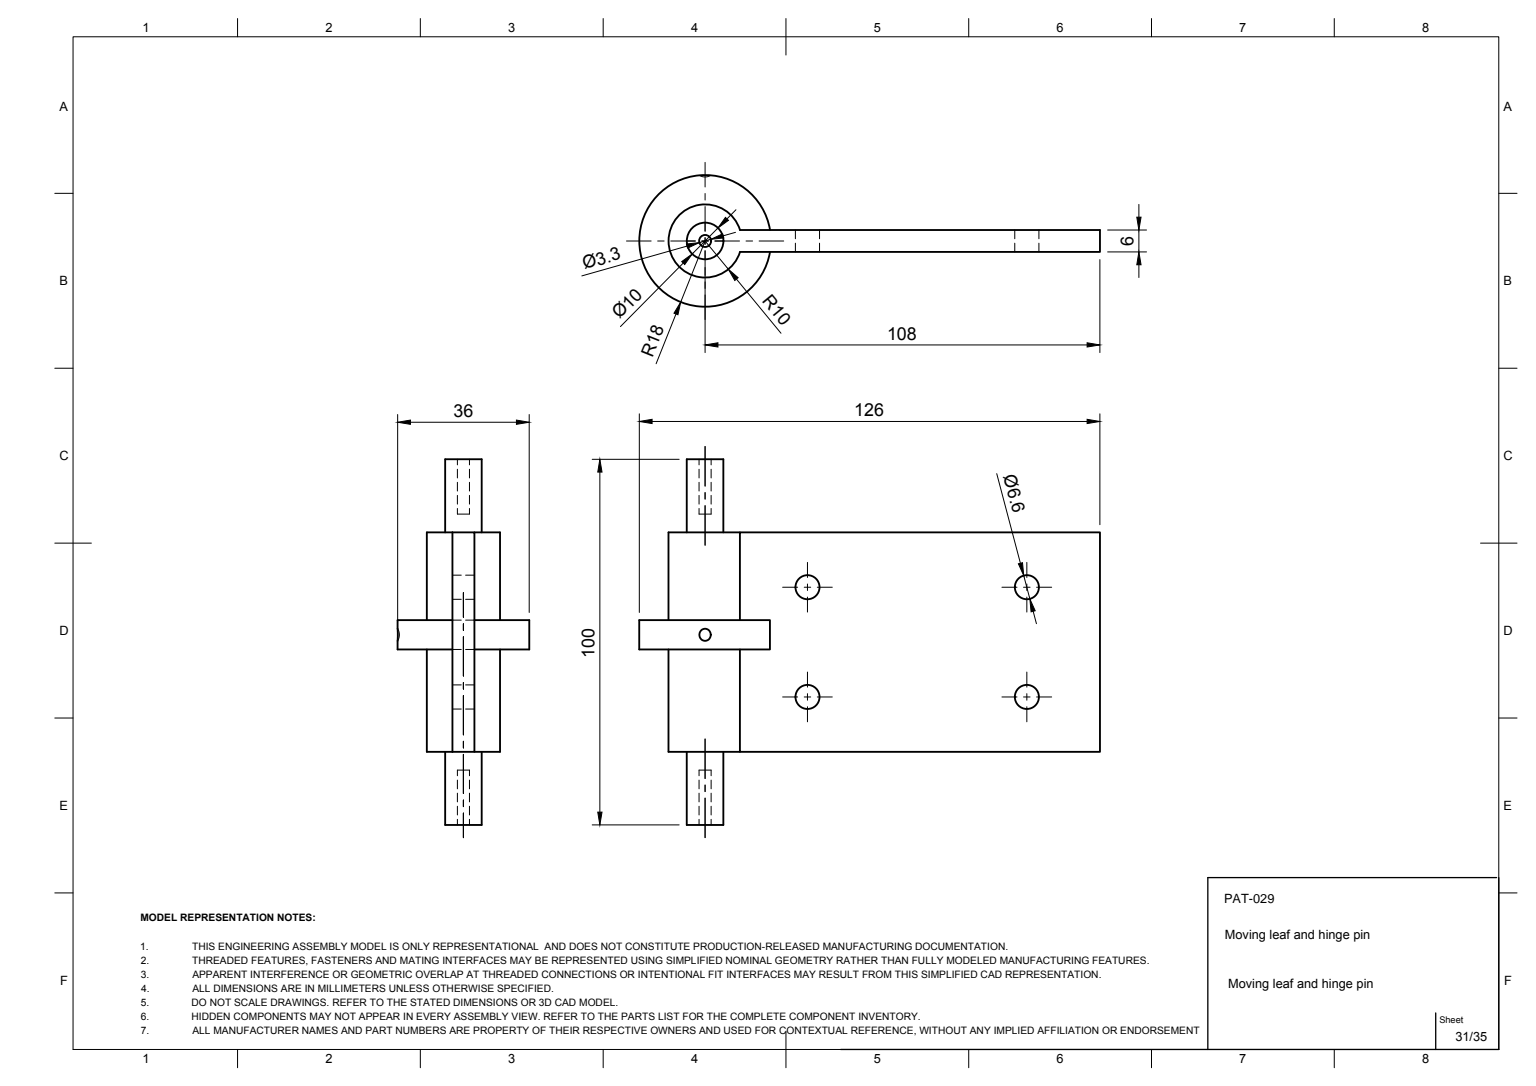
ISO-10303-21;
HEADER;
/* Generated by software containing ST-Developer
 * from STEP Tools, Inc. (www.steptools.com) 
 */

FILE_DESCRIPTION(
/* description */ ('Door-style hinge test fixture with detent'),
/* implementation_level */ '2;1');

FILE_NAME(
/* name */ 'Moving leaf and hinge pin.step',
/* time_stamp */ '2026-10-28T03:24:57-07:00',
/* author */ (''),
/* organization */ (''),
/* preprocessor_version */ 'ST-DEVELOPER v20.2',
/* originating_system */ 'Autodesk Translation Framework v15.17.0.0',
/* authorisation */ '');

FILE_SCHEMA (('AUTOMOTIVE_DESIGN { 1 0 10303 214 3 1 1 }'));
ENDSEC;

DATA;
#10=MECHANICAL_DESIGN_GEOMETRIC_PRESENTATION_REPRESENTATION('',(#356),#9813);
#240=B_SPLINE_CURVE_WITH_KNOTS('',3,(#9473,#9474,#9475,#9476,#9477,#9478,
#9479,#9480,#9481,#9482,#9483,#9484,#9485,#9486,#9487,#9488,#9489,#9490,
#9491,#9492,#9493,#9494,#9495,#9496,#9497,#9498,#9499,#9500,#9501,#9502,
#9503,#9504,#9505,#9506,#9507,#9508,#9509,#9510,#9511,#9512,#9513,#9514),
 .UNSPECIFIED.,.T.,.F.,(4,2,2,2,2,2,2,2,2,2,2,2,2,2,2,2,2,2,2,2,4),(0.,
0.0839475318916269,0.12592129783744,0.167895063783254,0.205982250035365,
0.244069436287477,0.282156622539588,0.320243808791699,0.362217574737513,
0.404191340683327,0.488138872574954,0.572086404466582,0.614060170412395,
0.656033936358209,0.694121122610321,0.732208308862432,0.770295495114543,
0.808382681366655,0.850356447312468,0.892330213258282,0.976277745149909),
 .UNSPECIFIED.);
#259=SPHERICAL_SURFACE('',#5643,0.3);
#285=SHAPE_REPRESENTATION_RELATIONSHIP('SRR','None',#9964,#316);
#316=ADVANCED_BREP_SHAPE_REPRESENTATION('',(#394),#9807);
#356=STYLED_ITEM('',(#10183),#394);
#394=MANIFOLD_SOLID_BREP('Body1',#4789);
#478=FACE_BOUND('',#1263,.T.);
#479=FACE_BOUND('',#1266,.T.);
#480=FACE_BOUND('',#1267,.T.);
#481=FACE_BOUND('',#1268,.T.);
#482=FACE_BOUND('',#1269,.T.);
#483=FACE_BOUND('',#1276,.T.);
#484=FACE_BOUND('',#1277,.T.);
#485=FACE_BOUND('',#1278,.T.);
#486=FACE_BOUND('',#1279,.T.);
#487=FACE_BOUND('',#1283,.T.);
#488=FACE_BOUND('',#1285,.T.);
#489=FACE_BOUND('',#1289,.T.);
#490=FACE_BOUND('',#1291,.T.);
#633=PLANE('',#5638);
#634=PLANE('',#5642);
#635=PLANE('',#5644);
#636=PLANE('',#5649);
#637=PLANE('',#5651);
#638=PLANE('',#5666);
#639=PLANE('',#5667);
#640=PLANE('',#5670);
#641=PLANE('',#5672);
#642=PLANE('',#5678);
#643=PLANE('',#5679);
#892=FACE_OUTER_BOUND('',#1256,.T.);
#893=FACE_OUTER_BOUND('',#1257,.T.);
#894=FACE_OUTER_BOUND('',#1258,.T.);
#895=FACE_OUTER_BOUND('',#1259,.T.);
#896=FACE_OUTER_BOUND('',#1260,.T.);
#897=FACE_OUTER_BOUND('',#1261,.T.);
#898=FACE_OUTER_BOUND('',#1262,.T.);
#899=FACE_OUTER_BOUND('',#1264,.T.);
#900=FACE_OUTER_BOUND('',#1265,.T.);
#901=FACE_OUTER_BOUND('',#1270,.T.);
#902=FACE_OUTER_BOUND('',#1271,.T.);
#903=FACE_OUTER_BOUND('',#1272,.T.);
#904=FACE_OUTER_BOUND('',#1273,.T.);
#905=FACE_OUTER_BOUND('',#1274,.T.);
#906=FACE_OUTER_BOUND('',#1275,.T.);
#907=FACE_OUTER_BOUND('',#1280,.T.);
#908=FACE_OUTER_BOUND('',#1281,.T.);
#909=FACE_OUTER_BOUND('',#1282,.T.);
#910=FACE_OUTER_BOUND('',#1284,.T.);
#911=FACE_OUTER_BOUND('',#1286,.T.);
#912=FACE_OUTER_BOUND('',#1287,.T.);
#913=FACE_OUTER_BOUND('',#1288,.T.);
#914=FACE_OUTER_BOUND('',#1290,.T.);
#1256=EDGE_LOOP('',(#4171,#4172,#4173,#4174));
#1257=EDGE_LOOP('',(#4175));
#1258=EDGE_LOOP('',(#4176,#4177,#4178,#4179));
#1259=EDGE_LOOP('',(#4180));
#1260=EDGE_LOOP('',(#4181));
#1261=EDGE_LOOP('',(#4182,#4183,#4184,#4185));
#1262=EDGE_LOOP('',(#4186,#4187,#4188,#4189));
#1263=EDGE_LOOP('',(#4190));
#1264=EDGE_LOOP('',(#4191,#4192,#4193,#4194));
#1265=EDGE_LOOP('',(#4195,#4196,#4197,#4198,#4199,#4200,#4201,#4202));
#1266=EDGE_LOOP('',(#4203));
#1267=EDGE_LOOP('',(#4204));
#1268=EDGE_LOOP('',(#4205));
#1269=EDGE_LOOP('',(#4206));
#1270=EDGE_LOOP('',(#4207,#4208,#4209,#4210));
#1271=EDGE_LOOP('',(#4211,#4212,#4213,#4214));
#1272=EDGE_LOOP('',(#4215,#4216,#4217,#4218));
#1273=EDGE_LOOP('',(#4219,#4220,#4221,#4222));
#1274=EDGE_LOOP('',(#4223,#4224,#4225,#4226));
#1275=EDGE_LOOP('',(#4227,#4228,#4229,#4230,#4231,#4232,#4233,#4234));
#1276=EDGE_LOOP('',(#4235));
#1277=EDGE_LOOP('',(#4236));
#1278=EDGE_LOOP('',(#4237));
#1279=EDGE_LOOP('',(#4238));
#1280=EDGE_LOOP('',(#4239,#4240,#4241,#4242));
#1281=EDGE_LOOP('',(#4243,#4244,#4245,#4246));
#1282=EDGE_LOOP('',(#4247,#4248,#4249,#4250));
#1283=EDGE_LOOP('',(#4251));
#1284=EDGE_LOOP('',(#4252,#4253,#4254,#4255));
#1285=EDGE_LOOP('',(#4256));
#1286=EDGE_LOOP('',(#4257,#4258,#4259,#4260));
#1287=EDGE_LOOP('',(#4261,#4262,#4263,#4264));
#1288=EDGE_LOOP('',(#4265));
#1289=EDGE_LOOP('',(#4266));
#1290=EDGE_LOOP('',(#4267));
#1291=EDGE_LOOP('',(#4268));
#1596=LINE('',#9461,#1916);
#1597=LINE('',#9468,#1917);
#1598=LINE('',#9518,#1918);
#1599=LINE('',#9522,#1919);
#1600=LINE('',#9526,#1920);
#1601=LINE('',#9528,#1921);
#1602=LINE('',#9532,#1922);
#1603=LINE('',#9534,#1923);
#1604=LINE('',#9538,#1924);
#1605=LINE('',#9540,#1925);
#1606=LINE('',#9542,#1926);
#1607=LINE('',#9544,#1927);
#1608=LINE('',#9545,#1928);
#1609=LINE('',#9556,#1929);
#1610=LINE('',#9560,#1930);
#1611=LINE('',#9564,#1931);
#1612=LINE('',#9568,#1932);
#1613=LINE('',#9572,#1933);
#1614=LINE('',#9576,#1934);
#1615=LINE('',#9578,#1935);
#1616=LINE('',#9580,#1936);
#1617=LINE('',#9581,#1937);
#1618=LINE('',#9583,#1938);
#1619=LINE('',#9584,#1939);
#1620=LINE('',#9595,#1940);
#1621=LINE('',#9600,#1941);
#1916=VECTOR('',#7011,0.165);
#1917=VECTOR('',#7020,0.165);
#1918=VECTOR('',#7029,1.);
#1919=VECTOR('',#7032,1.);
#1920=VECTOR('',#7037,1.);
#1921=VECTOR('',#7038,1.);
#1922=VECTOR('',#7043,1.);
#1923=VECTOR('',#7044,1.);
#1924=VECTOR('',#7049,1.);
#1925=VECTOR('',#7050,1.);
#1926=VECTOR('',#7051,1.);
#1927=VECTOR('',#7052,1.);
#1928=VECTOR('',#7053,1.);
#1929=VECTOR('',#7064,1.);
#1930=VECTOR('',#7069,0.33);
#1931=VECTOR('',#7074,0.33);
#1932=VECTOR('',#7079,0.33);
#1933=VECTOR('',#7084,0.33);
#1934=VECTOR('',#7089,1.);
#1935=VECTOR('',#7090,1.);
#1936=VECTOR('',#7091,1.);
#1937=VECTOR('',#7092,1.);
#1938=VECTOR('',#7095,1.);
#1939=VECTOR('',#7096,1.);
#1940=VECTOR('',#7111,0.5);
#1941=VECTOR('',#7118,0.5);
#2175=CIRCLE('',#5636,0.165);
#2176=CIRCLE('',#5637,0.165);
#2177=CIRCLE('',#5640,0.165);
#2178=CIRCLE('',#5641,0.165);
#2179=CIRCLE('',#5645,1.);
#2180=CIRCLE('',#5646,1.8);
#2181=CIRCLE('',#5648,1.8);
#2182=CIRCLE('',#5650,1.);
#2183=CIRCLE('',#5652,0.33);
#2184=CIRCLE('',#5653,0.33);
#2185=CIRCLE('',#5654,0.33);
#2186=CIRCLE('',#5655,0.33);
#2187=CIRCLE('',#5657,1.);
#2188=CIRCLE('',#5659,0.33);
#2189=CIRCLE('',#5661,0.33);
#2190=CIRCLE('',#5663,0.33);
#2191=CIRCLE('',#5665,0.33);
#2192=CIRCLE('',#5669,1.);
#2193=CIRCLE('',#5671,0.5);
#2194=CIRCLE('',#5673,0.5);
#2195=CIRCLE('',#5675,0.5);
#2196=CIRCLE('',#5677,0.5);
#2551=VERTEX_POINT('',#9458);
#2552=VERTEX_POINT('',#9460);
#2553=VERTEX_POINT('',#9465);
#2554=VERTEX_POINT('',#9467);
#2555=VERTEX_POINT('',#9472);
#2556=VERTEX_POINT('',#9516);
#2557=VERTEX_POINT('',#9517);
#2558=VERTEX_POINT('',#9519);
#2559=VERTEX_POINT('',#9521);
#2560=VERTEX_POINT('',#9525);
#2561=VERTEX_POINT('',#9527);
#2562=VERTEX_POINT('',#9531);
#2563=VERTEX_POINT('',#9533);
#2564=VERTEX_POINT('',#9537);
#2565=VERTEX_POINT('',#9539);
#2566=VERTEX_POINT('',#9541);
#2567=VERTEX_POINT('',#9543);
#2568=VERTEX_POINT('',#9546);
#2569=VERTEX_POINT('',#9548);
#2570=VERTEX_POINT('',#9550);
#2571=VERTEX_POINT('',#9552);
#2572=VERTEX_POINT('',#9555);
#2573=VERTEX_POINT('',#9559);
#2574=VERTEX_POINT('',#9563);
#2575=VERTEX_POINT('',#9567);
#2576=VERTEX_POINT('',#9571);
#2577=VERTEX_POINT('',#9575);
#2578=VERTEX_POINT('',#9577);
#2579=VERTEX_POINT('',#9579);
#2580=VERTEX_POINT('',#9588);
#2581=VERTEX_POINT('',#9591);
#2582=VERTEX_POINT('',#9594);
#2583=VERTEX_POINT('',#9598);
#3102=EDGE_CURVE('',#2551,#2551,#2175,.T.);
#3103=EDGE_CURVE('',#2551,#2552,#1596,.T.);
#3104=EDGE_CURVE('',#2552,#2552,#2176,.T.);
#3105=EDGE_CURVE('',#2553,#2553,#2177,.T.);
#3106=EDGE_CURVE('',#2553,#2554,#1597,.T.);
#3107=EDGE_CURVE('',#2554,#2554,#2178,.T.);
#3108=EDGE_CURVE('',#2555,#2555,#240,.T.);
#3109=EDGE_CURVE('',#2556,#2557,#1598,.T.);
#3110=EDGE_CURVE('',#2558,#2556,#2179,.T.);
#3111=EDGE_CURVE('',#2559,#2558,#1599,.T.);
#3112=EDGE_CURVE('',#2559,#2557,#2180,.T.);
#3113=EDGE_CURVE('',#2557,#2560,#1600,.T.);
#3114=EDGE_CURVE('',#2561,#2559,#1601,.T.);
#3115=EDGE_CURVE('',#2561,#2560,#2181,.T.);
#3116=EDGE_CURVE('',#2560,#2562,#1602,.T.);
#3117=EDGE_CURVE('',#2563,#2561,#1603,.T.);
#3118=EDGE_CURVE('',#2562,#2563,#2182,.T.);
#3119=EDGE_CURVE('',#2564,#2562,#1604,.T.);
#3120=EDGE_CURVE('',#2564,#2565,#1605,.T.);
#3121=EDGE_CURVE('',#2565,#2566,#1606,.T.);
#3122=EDGE_CURVE('',#2567,#2566,#1607,.T.);
#3123=EDGE_CURVE('',#2556,#2567,#1608,.T.);
#3124=EDGE_CURVE('',#2568,#2568,#2183,.T.);
#3125=EDGE_CURVE('',#2569,#2569,#2184,.T.);
#3126=EDGE_CURVE('',#2570,#2570,#2185,.T.);
#3127=EDGE_CURVE('',#2571,#2571,#2186,.T.);
#3128=EDGE_CURVE('',#2563,#2572,#1609,.T.);
#3129=EDGE_CURVE('',#2572,#2564,#2187,.T.);
#3130=EDGE_CURVE('',#2571,#2573,#1610,.T.);
#3131=EDGE_CURVE('',#2573,#2573,#2188,.T.);
#3132=EDGE_CURVE('',#2570,#2574,#1611,.T.);
#3133=EDGE_CURVE('',#2574,#2574,#2189,.T.);
#3134=EDGE_CURVE('',#2569,#2575,#1612,.T.);
#3135=EDGE_CURVE('',#2575,#2575,#2190,.T.);
#3136=EDGE_CURVE('',#2568,#2576,#1613,.T.);
#3137=EDGE_CURVE('',#2576,#2576,#2191,.T.);
#3138=EDGE_CURVE('',#2577,#2558,#1614,.T.);
#3139=EDGE_CURVE('',#2578,#2577,#1615,.T.);
#3140=EDGE_CURVE('',#2579,#2578,#1616,.T.);
#3141=EDGE_CURVE('',#2579,#2572,#1617,.T.);
#3142=EDGE_CURVE('',#2565,#2579,#1618,.T.);
#3143=EDGE_CURVE('',#2566,#2578,#1619,.T.);
#3144=EDGE_CURVE('',#2577,#2567,#2192,.T.);
#3145=EDGE_CURVE('',#2580,#2580,#2193,.T.);
#3146=EDGE_CURVE('',#2581,#2581,#2194,.T.);
#3147=EDGE_CURVE('',#2580,#2582,#1620,.T.);
#3148=EDGE_CURVE('',#2582,#2582,#2195,.T.);
#3149=EDGE_CURVE('',#2583,#2583,#2196,.T.);
#3150=EDGE_CURVE('',#2583,#2581,#1621,.T.);
#4171=ORIENTED_EDGE('',*,*,#3102,.F.);
#4172=ORIENTED_EDGE('',*,*,#3103,.T.);
#4173=ORIENTED_EDGE('',*,*,#3104,.F.);
#4174=ORIENTED_EDGE('',*,*,#3103,.F.);
#4175=ORIENTED_EDGE('',*,*,#3102,.T.);
#4176=ORIENTED_EDGE('',*,*,#3105,.F.);
#4177=ORIENTED_EDGE('',*,*,#3106,.T.);
#4178=ORIENTED_EDGE('',*,*,#3107,.T.);
#4179=ORIENTED_EDGE('',*,*,#3106,.F.);
#4180=ORIENTED_EDGE('',*,*,#3107,.F.);
#4181=ORIENTED_EDGE('',*,*,#3108,.F.);
#4182=ORIENTED_EDGE('',*,*,#3109,.F.);
#4183=ORIENTED_EDGE('',*,*,#3110,.F.);
#4184=ORIENTED_EDGE('',*,*,#3111,.F.);
#4185=ORIENTED_EDGE('',*,*,#3112,.T.);
#4186=ORIENTED_EDGE('',*,*,#3113,.F.);
#4187=ORIENTED_EDGE('',*,*,#3112,.F.);
#4188=ORIENTED_EDGE('',*,*,#3114,.F.);
#4189=ORIENTED_EDGE('',*,*,#3115,.T.);
#4190=ORIENTED_EDGE('',*,*,#3108,.T.);
#4191=ORIENTED_EDGE('',*,*,#3116,.F.);
#4192=ORIENTED_EDGE('',*,*,#3115,.F.);
#4193=ORIENTED_EDGE('',*,*,#3117,.F.);
#4194=ORIENTED_EDGE('',*,*,#3118,.F.);
#4195=ORIENTED_EDGE('',*,*,#3109,.T.);
#4196=ORIENTED_EDGE('',*,*,#3113,.T.);
#4197=ORIENTED_EDGE('',*,*,#3116,.T.);
#4198=ORIENTED_EDGE('',*,*,#3119,.F.);
#4199=ORIENTED_EDGE('',*,*,#3120,.T.);
#4200=ORIENTED_EDGE('',*,*,#3121,.T.);
#4201=ORIENTED_EDGE('',*,*,#3122,.F.);
#4202=ORIENTED_EDGE('',*,*,#3123,.F.);
#4203=ORIENTED_EDGE('',*,*,#3124,.T.);
#4204=ORIENTED_EDGE('',*,*,#3125,.T.);
#4205=ORIENTED_EDGE('',*,*,#3126,.T.);
#4206=ORIENTED_EDGE('',*,*,#3127,.T.);
#4207=ORIENTED_EDGE('',*,*,#3118,.T.);
#4208=ORIENTED_EDGE('',*,*,#3128,.T.);
#4209=ORIENTED_EDGE('',*,*,#3129,.T.);
#4210=ORIENTED_EDGE('',*,*,#3119,.T.);
#4211=ORIENTED_EDGE('',*,*,#3127,.F.);
#4212=ORIENTED_EDGE('',*,*,#3130,.T.);
#4213=ORIENTED_EDGE('',*,*,#3131,.F.);
#4214=ORIENTED_EDGE('',*,*,#3130,.F.);
#4215=ORIENTED_EDGE('',*,*,#3126,.F.);
#4216=ORIENTED_EDGE('',*,*,#3132,.T.);
#4217=ORIENTED_EDGE('',*,*,#3133,.F.);
#4218=ORIENTED_EDGE('',*,*,#3132,.F.);
#4219=ORIENTED_EDGE('',*,*,#3125,.F.);
#4220=ORIENTED_EDGE('',*,*,#3134,.T.);
#4221=ORIENTED_EDGE('',*,*,#3135,.F.);
#4222=ORIENTED_EDGE('',*,*,#3134,.F.);
#4223=ORIENTED_EDGE('',*,*,#3124,.F.);
#4224=ORIENTED_EDGE('',*,*,#3136,.T.);
#4225=ORIENTED_EDGE('',*,*,#3137,.F.);
#4226=ORIENTED_EDGE('',*,*,#3136,.F.);
#4227=ORIENTED_EDGE('',*,*,#3111,.T.);
#4228=ORIENTED_EDGE('',*,*,#3138,.F.);
#4229=ORIENTED_EDGE('',*,*,#3139,.F.);
#4230=ORIENTED_EDGE('',*,*,#3140,.F.);
#4231=ORIENTED_EDGE('',*,*,#3141,.T.);
#4232=ORIENTED_EDGE('',*,*,#3128,.F.);
#4233=ORIENTED_EDGE('',*,*,#3117,.T.);
#4234=ORIENTED_EDGE('',*,*,#3114,.T.);
#4235=ORIENTED_EDGE('',*,*,#3131,.T.);
#4236=ORIENTED_EDGE('',*,*,#3133,.T.);
#4237=ORIENTED_EDGE('',*,*,#3135,.T.);
#4238=ORIENTED_EDGE('',*,*,#3137,.T.);
#4239=ORIENTED_EDGE('',*,*,#3142,.T.);
#4240=ORIENTED_EDGE('',*,*,#3140,.T.);
#4241=ORIENTED_EDGE('',*,*,#3143,.F.);
#4242=ORIENTED_EDGE('',*,*,#3121,.F.);
#4243=ORIENTED_EDGE('',*,*,#3110,.T.);
#4244=ORIENTED_EDGE('',*,*,#3123,.T.);
#4245=ORIENTED_EDGE('',*,*,#3144,.F.);
#4246=ORIENTED_EDGE('',*,*,#3138,.T.);
#4247=ORIENTED_EDGE('',*,*,#3129,.F.);
#4248=ORIENTED_EDGE('',*,*,#3141,.F.);
#4249=ORIENTED_EDGE('',*,*,#3142,.F.);
#4250=ORIENTED_EDGE('',*,*,#3120,.F.);
#4251=ORIENTED_EDGE('',*,*,#3145,.F.);
#4252=ORIENTED_EDGE('',*,*,#3144,.T.);
#4253=ORIENTED_EDGE('',*,*,#3122,.T.);
#4254=ORIENTED_EDGE('',*,*,#3143,.T.);
#4255=ORIENTED_EDGE('',*,*,#3139,.T.);
#4256=ORIENTED_EDGE('',*,*,#3146,.F.);
#4257=ORIENTED_EDGE('',*,*,#3145,.T.);
#4258=ORIENTED_EDGE('',*,*,#3147,.T.);
#4259=ORIENTED_EDGE('',*,*,#3148,.T.);
#4260=ORIENTED_EDGE('',*,*,#3147,.F.);
#4261=ORIENTED_EDGE('',*,*,#3149,.F.);
#4262=ORIENTED_EDGE('',*,*,#3150,.T.);
#4263=ORIENTED_EDGE('',*,*,#3146,.T.);
#4264=ORIENTED_EDGE('',*,*,#3150,.F.);
#4265=ORIENTED_EDGE('',*,*,#3149,.T.);
#4266=ORIENTED_EDGE('',*,*,#3104,.T.);
#4267=ORIENTED_EDGE('',*,*,#3148,.F.);
#4268=ORIENTED_EDGE('',*,*,#3105,.T.);
#4447=CYLINDRICAL_SURFACE('',#5635,0.165);
#4448=CYLINDRICAL_SURFACE('',#5639,0.165);
#4449=CYLINDRICAL_SURFACE('',#5647,1.8);
#4450=CYLINDRICAL_SURFACE('',#5656,1.);
#4451=CYLINDRICAL_SURFACE('',#5658,0.33);
#4452=CYLINDRICAL_SURFACE('',#5660,0.33);
#4453=CYLINDRICAL_SURFACE('',#5662,0.33);
#4454=CYLINDRICAL_SURFACE('',#5664,0.33);
#4455=CYLINDRICAL_SURFACE('',#5668,1.);
#4456=CYLINDRICAL_SURFACE('',#5674,0.5);
#4457=CYLINDRICAL_SURFACE('',#5676,0.5);
#4697=ADVANCED_FACE('',(#892),#4447,.F.);
#4698=ADVANCED_FACE('',(#893),#633,.T.);
#4699=ADVANCED_FACE('',(#894),#4448,.F.);
#4700=ADVANCED_FACE('',(#895),#634,.F.);
#4701=ADVANCED_FACE('',(#896),#259,.F.);
#4702=ADVANCED_FACE('',(#897),#635,.T.);
#4703=ADVANCED_FACE('',(#898,#478),#4449,.T.);
#4704=ADVANCED_FACE('',(#899),#636,.F.);
#4705=ADVANCED_FACE('',(#900,#479,#480,#481,#482),#637,.T.);
#4706=ADVANCED_FACE('',(#901),#4450,.T.);
#4707=ADVANCED_FACE('',(#902),#4451,.F.);
#4708=ADVANCED_FACE('',(#903),#4452,.F.);
#4709=ADVANCED_FACE('',(#904),#4453,.F.);
#4710=ADVANCED_FACE('',(#905),#4454,.F.);
#4711=ADVANCED_FACE('',(#906,#483,#484,#485,#486),#638,.T.);
#4712=ADVANCED_FACE('',(#907),#639,.T.);
#4713=ADVANCED_FACE('',(#908),#4455,.T.);
#4714=ADVANCED_FACE('',(#909,#487),#640,.F.);
#4715=ADVANCED_FACE('',(#910,#488),#641,.T.);
#4716=ADVANCED_FACE('',(#911),#4456,.T.);
#4717=ADVANCED_FACE('',(#912),#4457,.T.);
#4718=ADVANCED_FACE('',(#913,#489),#642,.T.);
#4719=ADVANCED_FACE('',(#914,#490),#643,.F.);
#4789=CLOSED_SHELL('',(#4697,#4698,#4699,#4700,#4701,#4702,#4703,#4704,
#4705,#4706,#4707,#4708,#4709,#4710,#4711,#4712,#4713,#4714,#4715,#4716,
#4717,#4718,#4719));
#5634=AXIS2_PLACEMENT_3D('',#9456,#7005,#7006);
#5635=AXIS2_PLACEMENT_3D('',#9457,#7007,#7008);
#5636=AXIS2_PLACEMENT_3D('',#9459,#7009,#7010);
#5637=AXIS2_PLACEMENT_3D('',#9462,#7012,#7013);
#5638=AXIS2_PLACEMENT_3D('',#9463,#7014,#7015);
#5639=AXIS2_PLACEMENT_3D('',#9464,#7016,#7017);
#5640=AXIS2_PLACEMENT_3D('',#9466,#7018,#7019);
#5641=AXIS2_PLACEMENT_3D('',#9469,#7021,#7022);
#5642=AXIS2_PLACEMENT_3D('',#9470,#7023,#7024);
#5643=AXIS2_PLACEMENT_3D('',#9471,#7025,#7026);
#5644=AXIS2_PLACEMENT_3D('',#9515,#7027,#7028);
#5645=AXIS2_PLACEMENT_3D('',#9520,#7030,#7031);
#5646=AXIS2_PLACEMENT_3D('',#9523,#7033,#7034);
#5647=AXIS2_PLACEMENT_3D('',#9524,#7035,#7036);
#5648=AXIS2_PLACEMENT_3D('',#9529,#7039,#7040);
#5649=AXIS2_PLACEMENT_3D('',#9530,#7041,#7042);
#5650=AXIS2_PLACEMENT_3D('',#9535,#7045,#7046);
#5651=AXIS2_PLACEMENT_3D('',#9536,#7047,#7048);
#5652=AXIS2_PLACEMENT_3D('',#9547,#7054,#7055);
#5653=AXIS2_PLACEMENT_3D('',#9549,#7056,#7057);
#5654=AXIS2_PLACEMENT_3D('',#9551,#7058,#7059);
#5655=AXIS2_PLACEMENT_3D('',#9553,#7060,#7061);
#5656=AXIS2_PLACEMENT_3D('',#9554,#7062,#7063);
#5657=AXIS2_PLACEMENT_3D('',#9557,#7065,#7066);
#5658=AXIS2_PLACEMENT_3D('',#9558,#7067,#7068);
#5659=AXIS2_PLACEMENT_3D('',#9561,#7070,#7071);
#5660=AXIS2_PLACEMENT_3D('',#9562,#7072,#7073);
#5661=AXIS2_PLACEMENT_3D('',#9565,#7075,#7076);
#5662=AXIS2_PLACEMENT_3D('',#9566,#7077,#7078);
#5663=AXIS2_PLACEMENT_3D('',#9569,#7080,#7081);
#5664=AXIS2_PLACEMENT_3D('',#9570,#7082,#7083);
#5665=AXIS2_PLACEMENT_3D('',#9573,#7085,#7086);
#5666=AXIS2_PLACEMENT_3D('',#9574,#7087,#7088);
#5667=AXIS2_PLACEMENT_3D('',#9582,#7093,#7094);
#5668=AXIS2_PLACEMENT_3D('',#9585,#7097,#7098);
#5669=AXIS2_PLACEMENT_3D('',#9586,#7099,#7100);
#5670=AXIS2_PLACEMENT_3D('',#9587,#7101,#7102);
#5671=AXIS2_PLACEMENT_3D('',#9589,#7103,#7104);
#5672=AXIS2_PLACEMENT_3D('',#9590,#7105,#7106);
#5673=AXIS2_PLACEMENT_3D('',#9592,#7107,#7108);
#5674=AXIS2_PLACEMENT_3D('',#9593,#7109,#7110);
#5675=AXIS2_PLACEMENT_3D('',#9596,#7112,#7113);
#5676=AXIS2_PLACEMENT_3D('',#9597,#7114,#7115);
#5677=AXIS2_PLACEMENT_3D('',#9599,#7116,#7117);
#5678=AXIS2_PLACEMENT_3D('',#9601,#7119,#7120);
#5679=AXIS2_PLACEMENT_3D('',#9602,#7121,#7122);
#7005=DIRECTION('axis',(0.,0.,1.));
#7006=DIRECTION('refdir',(1.,0.,0.));
#7007=DIRECTION('center_axis',(0.,0.,1.));
#7008=DIRECTION('ref_axis',(1.,0.,0.));
#7009=DIRECTION('center_axis',(0.,0.,1.));
#7010=DIRECTION('ref_axis',(1.,0.,0.));
#7011=DIRECTION('',(0.,0.,1.));
#7012=DIRECTION('center_axis',(0.,0.,-1.));
#7013=DIRECTION('ref_axis',(1.,0.,0.));
#7014=DIRECTION('center_axis',(0.,0.,1.));
#7015=DIRECTION('ref_axis',(1.,0.,0.));
#7016=DIRECTION('center_axis',(0.,0.,1.));
#7017=DIRECTION('ref_axis',(1.,0.,0.));
#7018=DIRECTION('center_axis',(0.,0.,1.));
#7019=DIRECTION('ref_axis',(1.,0.,0.));
#7020=DIRECTION('',(0.,0.,1.));
#7021=DIRECTION('center_axis',(0.,0.,1.));
#7022=DIRECTION('ref_axis',(1.,0.,0.));
#7023=DIRECTION('center_axis',(0.,0.,1.));
#7024=DIRECTION('ref_axis',(1.,0.,0.));
#7025=DIRECTION('center_axis',(6.12323399573677E-17,0.,1.));
#7026=DIRECTION('ref_axis',(1.,0.,0.));
#7027=DIRECTION('center_axis',(0.,0.,1.));
#7028=DIRECTION('ref_axis',(1.,0.,0.));
#7029=DIRECTION('',(1.,0.,0.));
#7030=DIRECTION('center_axis',(0.,0.,1.));
#7031=DIRECTION('ref_axis',(1.,0.,0.));
#7032=DIRECTION('',(-1.,0.,0.));
#7033=DIRECTION('center_axis',(0.,0.,1.));
#7034=DIRECTION('ref_axis',(1.,0.,0.));
#7035=DIRECTION('center_axis',(0.,0.,1.));
#7036=DIRECTION('ref_axis',(-1.,-1.22464679914735E-16,0.));
#7037=DIRECTION('',(0.,0.,-1.));
#7038=DIRECTION('',(0.,0.,1.));
#7039=DIRECTION('center_axis',(0.,0.,1.));
#7040=DIRECTION('ref_axis',(1.,0.,0.));
#7041=DIRECTION('center_axis',(0.,0.,1.));
#7042=DIRECTION('ref_axis',(1.,0.,0.));
#7043=DIRECTION('',(-1.,0.,0.));
#7044=DIRECTION('',(1.,0.,0.));
#7045=DIRECTION('center_axis',(0.,0.,-1.));
#7046=DIRECTION('ref_axis',(1.,0.,0.));
#7047=DIRECTION('center_axis',(0.,-1.,0.));
#7048=DIRECTION('ref_axis',(1.,0.,0.));
#7049=DIRECTION('',(0.,0.,1.));
#7050=DIRECTION('',(1.,0.,0.));
#7051=DIRECTION('',(0.,0.,1.));
#7052=DIRECTION('',(1.,0.,0.));
#7053=DIRECTION('',(0.,0.,1.));
#7054=DIRECTION('center_axis',(0.,1.,0.));
#7055=DIRECTION('ref_axis',(1.,0.,0.));
#7056=DIRECTION('center_axis',(0.,1.,0.));
#7057=DIRECTION('ref_axis',(1.,0.,0.));
#7058=DIRECTION('center_axis',(0.,1.,0.));
#7059=DIRECTION('ref_axis',(1.,0.,0.));
#7060=DIRECTION('center_axis',(0.,1.,0.));
#7061=DIRECTION('ref_axis',(1.,0.,0.));
#7062=DIRECTION('center_axis',(0.,0.,1.));
#7063=DIRECTION('ref_axis',(-1.,1.22464679914735E-16,0.));
#7064=DIRECTION('',(0.,0.,-1.));
#7065=DIRECTION('center_axis',(0.,0.,1.));
#7066=DIRECTION('ref_axis',(1.,0.,0.));
#7067=DIRECTION('center_axis',(0.,1.,0.));
#7068=DIRECTION('ref_axis',(1.,0.,0.));
#7069=DIRECTION('',(0.,1.,0.));
#7070=DIRECTION('center_axis',(0.,-1.,0.));
#7071=DIRECTION('ref_axis',(1.,0.,0.));
#7072=DIRECTION('center_axis',(0.,1.,0.));
#7073=DIRECTION('ref_axis',(1.,0.,0.));
#7074=DIRECTION('',(0.,1.,0.));
#7075=DIRECTION('center_axis',(0.,-1.,0.));
#7076=DIRECTION('ref_axis',(1.,0.,0.));
#7077=DIRECTION('center_axis',(0.,1.,0.));
#7078=DIRECTION('ref_axis',(1.,0.,0.));
#7079=DIRECTION('',(0.,1.,0.));
#7080=DIRECTION('center_axis',(0.,-1.,0.));
#7081=DIRECTION('ref_axis',(1.,0.,0.));
#7082=DIRECTION('center_axis',(0.,1.,0.));
#7083=DIRECTION('ref_axis',(1.,0.,0.));
#7084=DIRECTION('',(0.,1.,0.));
#7085=DIRECTION('center_axis',(0.,-1.,0.));
#7086=DIRECTION('ref_axis',(1.,0.,0.));
#7087=DIRECTION('center_axis',(0.,1.,0.));
#7088=DIRECTION('ref_axis',(-1.,0.,0.));
#7089=DIRECTION('',(0.,0.,-1.));
#7090=DIRECTION('',(-1.,0.,0.));
#7091=DIRECTION('',(0.,0.,1.));
#7092=DIRECTION('',(-1.,0.,0.));
#7093=DIRECTION('center_axis',(1.,0.,0.));
#7094=DIRECTION('ref_axis',(0.,1.,0.));
#7095=DIRECTION('',(0.,1.,0.));
#7096=DIRECTION('',(0.,1.,0.));
#7097=DIRECTION('center_axis',(0.,0.,1.));
#7098=DIRECTION('ref_axis',(-1.,1.22464679914735E-16,0.));
#7099=DIRECTION('center_axis',(0.,0.,1.));
#7100=DIRECTION('ref_axis',(1.,0.,0.));
#7101=DIRECTION('center_axis',(0.,0.,1.));
#7102=DIRECTION('ref_axis',(1.,0.,0.));
#7103=DIRECTION('center_axis',(0.,0.,-1.));
#7104=DIRECTION('ref_axis',(1.,0.,0.));
#7105=DIRECTION('center_axis',(0.,0.,1.));
#7106=DIRECTION('ref_axis',(1.,0.,0.));
#7107=DIRECTION('center_axis',(0.,0.,1.));
#7108=DIRECTION('ref_axis',(1.,0.,0.));
#7109=DIRECTION('center_axis',(0.,0.,1.));
#7110=DIRECTION('ref_axis',(1.,0.,0.));
#7111=DIRECTION('',(0.,0.,-1.));
#7112=DIRECTION('center_axis',(0.,0.,1.));
#7113=DIRECTION('ref_axis',(1.,0.,0.));
#7114=DIRECTION('center_axis',(0.,0.,1.));
#7115=DIRECTION('ref_axis',(1.,0.,0.));
#7116=DIRECTION('center_axis',(0.,0.,1.));
#7117=DIRECTION('ref_axis',(1.,0.,0.));
#7118=DIRECTION('',(0.,0.,-1.));
#7119=DIRECTION('center_axis',(0.,0.,1.));
#7120=DIRECTION('ref_axis',(1.,0.,0.));
#7121=DIRECTION('center_axis',(0.,0.,1.));
#7122=DIRECTION('ref_axis',(1.,0.,0.));
#9456=CARTESIAN_POINT('',(0.,0.,0.));
#9457=CARTESIAN_POINT('Origin',(0.,0.,10.5));
#9458=CARTESIAN_POINT('',(-0.165,-2.02066721859313E-17,10.5));
#9459=CARTESIAN_POINT('Origin',(0.,0.,10.5));
#9460=CARTESIAN_POINT('',(-0.165,2.02066721859313E-17,12.));
#9461=CARTESIAN_POINT('',(-0.165,-2.02066721859313E-17,10.5));
#9462=CARTESIAN_POINT('Origin',(0.,0.,12.));
#9463=CARTESIAN_POINT('Origin',(0.,0.,10.5));
#9464=CARTESIAN_POINT('Origin',(0.,0.,1.9));
#9465=CARTESIAN_POINT('',(-0.165,-2.02066721859313E-17,2.));
#9466=CARTESIAN_POINT('Origin',(0.,0.,2.));
#9467=CARTESIAN_POINT('',(-0.165,-2.02066721859313E-17,3.5));
#9468=CARTESIAN_POINT('',(-0.165,-2.02066721859313E-17,1.9));
#9469=CARTESIAN_POINT('Origin',(0.,0.,3.5));
#9470=CARTESIAN_POINT('Origin',(0.,0.,3.5));
#9471=CARTESIAN_POINT('Origin',(0.,-2.05,7.2));
#9472=CARTESIAN_POINT('',(0.155246105783993,-1.79329268292683,7.2));
#9473=CARTESIAN_POINT('Ctrl Pts',(0.155246105783993,-1.79329268292683,7.2));
#9474=CARTESIAN_POINT('Ctrl Pts',(0.155246105783993,-1.79329268292683,7.17201748936946));
#9475=CARTESIAN_POINT('Ctrl Pts',(0.148285663496836,-1.79393443972947,7.14272186726396));
#9476=CARTESIAN_POINT('Ctrl Pts',(0.127697249529238,-1.79547787365052,7.1044926805215));
#9477=CARTESIAN_POINT('Ctrl Pts',(0.119189936856738,-1.79607670590828,7.0926589910604));
#9478=CARTESIAN_POINT('Ctrl Pts',(0.0995353781147738,-1.79727260133503,
7.07183236368701));
#9479=CARTESIAN_POINT('Ctrl Pts',(0.08838803635753,-1.7978684994743,7.06283944919615));
#9480=CARTESIAN_POINT('Ctrl Pts',(0.0655526842737879,-1.79883881216911,
7.04906264597394));
#9481=CARTESIAN_POINT('Ctrl Pts',(0.0528849064848421,-1.79927148532923,
7.04338913442002));
#9482=CARTESIAN_POINT('Ctrl Pts',(0.0264570277515568,-1.79985408312092,
7.03594022256534));
#9483=CARTESIAN_POINT('Ctrl Pts',(0.0126957287507039,-1.8,7.03416876048223));
#9484=CARTESIAN_POINT('Ctrl Pts',(-0.0126957287507037,-1.8,7.03416876048223));
#9485=CARTESIAN_POINT('Ctrl Pts',(-0.0264570277515565,-1.79985408312092,
7.03594022256534));
#9486=CARTESIAN_POINT('Ctrl Pts',(-0.0528849064848418,-1.79927148532923,
7.04338913442002));
#9487=CARTESIAN_POINT('Ctrl Pts',(-0.0655526842737877,-1.79883881216911,
7.04906264597394));
#9488=CARTESIAN_POINT('Ctrl Pts',(-0.0883880363575299,-1.7978684994743,
7.06283944919615));
#9489=CARTESIAN_POINT('Ctrl Pts',(-0.0995353781147733,-1.79727260133503,
7.07183236368701));
#9490=CARTESIAN_POINT('Ctrl Pts',(-0.119189936856738,-1.79607670590828,
7.0926589910604));
#9491=CARTESIAN_POINT('Ctrl Pts',(-0.127697249529239,-1.79547787365052,
7.1044926805215));
#9492=CARTESIAN_POINT('Ctrl Pts',(-0.148285663496837,-1.79393443972947,
7.14272186726397));
#9493=CARTESIAN_POINT('Ctrl Pts',(-0.155246105783993,-1.79329268292683,
7.17201748936946));
#9494=CARTESIAN_POINT('Ctrl Pts',(-0.155246105783993,-1.79329268292683,
7.22798251063054));
#9495=CARTESIAN_POINT('Ctrl Pts',(-0.148285663496836,-1.79393443972947,
7.25727813273604));
#9496=CARTESIAN_POINT('Ctrl Pts',(-0.127697249529237,-1.79547787365052,
7.2955073194785));
#9497=CARTESIAN_POINT('Ctrl Pts',(-0.119189936856737,-1.79607670590828,
7.3073410089396));
#9498=CARTESIAN_POINT('Ctrl Pts',(-0.0995353781147728,-1.79727260133503,
7.32816763631299));
#9499=CARTESIAN_POINT('Ctrl Pts',(-0.0883880363575299,-1.7978684994743,
7.33716055080385));
#9500=CARTESIAN_POINT('Ctrl Pts',(-0.0655526842737877,-1.79883881216911,
7.35093735402606));
#9501=CARTESIAN_POINT('Ctrl Pts',(-0.0528849064848417,-1.79927148532923,
7.35661086557998));
#9502=CARTESIAN_POINT('Ctrl Pts',(-0.0264570277515566,-1.79985408312092,
7.36405977743466));
#9503=CARTESIAN_POINT('Ctrl Pts',(-0.0126957287507037,-1.8,7.36583123951777));
#9504=CARTESIAN_POINT('Ctrl Pts',(0.0126957287507039,-1.8,7.36583123951777));
#9505=CARTESIAN_POINT('Ctrl Pts',(0.0264570277515567,-1.79985408312092,
7.36405977743466));
#9506=CARTESIAN_POINT('Ctrl Pts',(0.0528849064848419,-1.79927148532923,
7.35661086557998));
#9507=CARTESIAN_POINT('Ctrl Pts',(0.0655526842737879,-1.79883881216911,
7.35093735402606));
#9508=CARTESIAN_POINT('Ctrl Pts',(0.08838803635753,-1.7978684994743,7.33716055080385));
#9509=CARTESIAN_POINT('Ctrl Pts',(0.0995353781147734,-1.79727260133503,
7.32816763631299));
#9510=CARTESIAN_POINT('Ctrl Pts',(0.119189936856738,-1.79607670590828,7.3073410089396));
#9511=CARTESIAN_POINT('Ctrl Pts',(0.127697249529238,-1.79547787365052,7.2955073194785));
#9512=CARTESIAN_POINT('Ctrl Pts',(0.148285663496836,-1.79393443972947,7.25727813273604));
#9513=CARTESIAN_POINT('Ctrl Pts',(0.155246105783993,-1.79329268292683,7.22798251063054));
#9514=CARTESIAN_POINT('Ctrl Pts',(0.155246105783993,-1.79329268292683,7.2));
#9515=CARTESIAN_POINT('Origin',(0.,0.,7.6));
#9516=CARTESIAN_POINT('',(0.953939201416946,-0.3,7.6));
#9517=CARTESIAN_POINT('',(1.77482393492988,-0.3,7.6));
#9518=CARTESIAN_POINT('',(0.4,-0.3,7.6));
#9519=CARTESIAN_POINT('',(0.953939201416946,0.3,7.6));
#9520=CARTESIAN_POINT('Origin',(0.,0.,7.6));
#9521=CARTESIAN_POINT('',(1.77482393492988,0.3,7.6));
#9522=CARTESIAN_POINT('',(5.4,0.3,7.6));
#9523=CARTESIAN_POINT('Origin',(0.,0.,7.6));
#9524=CARTESIAN_POINT('Origin',(0.,0.,6.8));
#9525=CARTESIAN_POINT('',(1.77482393492988,-0.3,6.8));
#9526=CARTESIAN_POINT('',(1.77482393492988,-0.3,6.8));
#9527=CARTESIAN_POINT('',(1.77482393492988,0.3,6.8));
#9528=CARTESIAN_POINT('',(1.77482393492988,0.3,6.8));
#9529=CARTESIAN_POINT('Origin',(0.,0.,6.8));
#9530=CARTESIAN_POINT('Origin',(0.,0.,6.8));
#9531=CARTESIAN_POINT('',(0.953939201416946,-0.3,6.8));
#9532=CARTESIAN_POINT('',(0.4,-0.3,6.8));
#9533=CARTESIAN_POINT('',(0.953939201416946,0.3,6.8));
#9534=CARTESIAN_POINT('',(5.4,0.3,6.8));
#9535=CARTESIAN_POINT('Origin',(0.,0.,6.8));
#9536=CARTESIAN_POINT('Origin',(0.8,-0.3,4.));
#9537=CARTESIAN_POINT('',(0.953939201416946,-0.3,4.));
#9538=CARTESIAN_POINT('',(0.953939201416946,-0.3,4.));
#9539=CARTESIAN_POINT('',(10.8,-0.3,4.));
#9540=CARTESIAN_POINT('',(0.8,-0.3,4.));
#9541=CARTESIAN_POINT('',(10.8,-0.3,10.));
#9542=CARTESIAN_POINT('',(10.8,-0.3,4.));
#9543=CARTESIAN_POINT('',(0.953939201416946,-0.3,10.));
#9544=CARTESIAN_POINT('',(0.8,-0.3,10.));
#9545=CARTESIAN_POINT('',(0.953939201416946,-0.3,4.));
#9546=CARTESIAN_POINT('',(8.47,-0.3,8.5));
#9547=CARTESIAN_POINT('Origin',(8.8,-0.3,8.5));
#9548=CARTESIAN_POINT('',(2.47,-0.3,5.5));
#9549=CARTESIAN_POINT('Origin',(2.8,-0.3,5.5));
#9550=CARTESIAN_POINT('',(2.47,-0.3,8.5));
#9551=CARTESIAN_POINT('Origin',(2.8,-0.3,8.5));
#9552=CARTESIAN_POINT('',(8.47,-0.3,5.5));
#9553=CARTESIAN_POINT('Origin',(8.8,-0.3,5.5));
#9554=CARTESIAN_POINT('Origin',(0.,0.,4.));
#9555=CARTESIAN_POINT('',(0.953939201416946,0.3,4.));
#9556=CARTESIAN_POINT('',(0.953939201416946,0.3,4.));
#9557=CARTESIAN_POINT('Origin',(0.,0.,4.));
#9558=CARTESIAN_POINT('Origin',(8.8,-0.4,5.5));
#9559=CARTESIAN_POINT('',(8.47,0.3,5.5));
#9560=CARTESIAN_POINT('',(8.47,-0.4,5.5));
#9561=CARTESIAN_POINT('Origin',(8.8,0.3,5.5));
#9562=CARTESIAN_POINT('Origin',(2.8,-0.4,8.5));
#9563=CARTESIAN_POINT('',(2.47,0.3,8.5));
#9564=CARTESIAN_POINT('',(2.47,-0.4,8.5));
#9565=CARTESIAN_POINT('Origin',(2.8,0.3,8.5));
#9566=CARTESIAN_POINT('Origin',(2.8,-0.4,5.5));
#9567=CARTESIAN_POINT('',(2.47,0.3,5.5));
#9568=CARTESIAN_POINT('',(2.47,-0.4,5.5));
#9569=CARTESIAN_POINT('Origin',(2.8,0.3,5.5));
#9570=CARTESIAN_POINT('Origin',(8.8,-0.4,8.5));
#9571=CARTESIAN_POINT('',(8.47,0.3,8.5));
#9572=CARTESIAN_POINT('',(8.47,-0.4,8.5));
#9573=CARTESIAN_POINT('Origin',(8.8,0.3,8.5));
#9574=CARTESIAN_POINT('Origin',(10.8,0.3,4.));
#9575=CARTESIAN_POINT('',(0.953939201416946,0.3,10.));
#9576=CARTESIAN_POINT('',(0.953939201416946,0.3,4.));
#9577=CARTESIAN_POINT('',(10.8,0.3,10.));
#9578=CARTESIAN_POINT('',(10.8,0.3,10.));
#9579=CARTESIAN_POINT('',(10.8,0.3,4.));
#9580=CARTESIAN_POINT('',(10.8,0.3,4.));
#9581=CARTESIAN_POINT('',(10.8,0.3,4.));
#9582=CARTESIAN_POINT('Origin',(10.8,-0.3,4.));
#9583=CARTESIAN_POINT('',(10.8,-0.3,4.));
#9584=CARTESIAN_POINT('',(10.8,-0.3,10.));
#9585=CARTESIAN_POINT('Origin',(0.,0.,4.));
#9586=CARTESIAN_POINT('Origin',(0.,0.,10.));
#9587=CARTESIAN_POINT('Origin',(0.,0.,4.));
#9588=CARTESIAN_POINT('',(-0.5,6.12323399573677E-17,4.));
#9589=CARTESIAN_POINT('Origin',(0.,0.,4.));
#9590=CARTESIAN_POINT('Origin',(0.,0.,10.));
#9591=CARTESIAN_POINT('',(-0.5,-6.12323399573677E-17,10.));
#9592=CARTESIAN_POINT('Origin',(0.,0.,10.));
#9593=CARTESIAN_POINT('Origin',(0.,0.,2.));
#9594=CARTESIAN_POINT('',(-0.5,-6.12323399573677E-17,2.));
#9595=CARTESIAN_POINT('',(-0.5,-6.12323399573677E-17,2.));
#9596=CARTESIAN_POINT('Origin',(0.,0.,2.));
#9597=CARTESIAN_POINT('Origin',(0.,0.,2.));
#9598=CARTESIAN_POINT('',(-0.5,-6.12323399573677E-17,12.));
#9599=CARTESIAN_POINT('Origin',(0.,0.,12.));
#9600=CARTESIAN_POINT('',(-0.5,-6.12323399573677E-17,2.));
#9601=CARTESIAN_POINT('Origin',(0.,0.,12.));
#9602=CARTESIAN_POINT('Origin',(0.,0.,2.));
#9771=UNCERTAINTY_MEASURE_WITH_UNIT(LENGTH_MEASURE(0.001),#9814,
'DISTANCE_ACCURACY_VALUE',
'Maximum model space distance between geometric entities at asserted c
onnectivities');
#9777=UNCERTAINTY_MEASURE_WITH_UNIT(LENGTH_MEASURE(0.001),#9814,
'DISTANCE_ACCURACY_VALUE',
'Maximum model space distance between geometric entities at asserted c
onnectivities');
#9807=(
GEOMETRIC_REPRESENTATION_CONTEXT(3)
GLOBAL_UNCERTAINTY_ASSIGNED_CONTEXT((#9771))
GLOBAL_UNIT_ASSIGNED_CONTEXT((#9814,#9816,#9817))
REPRESENTATION_CONTEXT('','3D')
);
#9813=(
GEOMETRIC_REPRESENTATION_CONTEXT(3)
GLOBAL_UNCERTAINTY_ASSIGNED_CONTEXT((#9777))
GLOBAL_UNIT_ASSIGNED_CONTEXT((#9814,#9816,#9817))
REPRESENTATION_CONTEXT('','3D')
);
#9814=(
LENGTH_UNIT()
NAMED_UNIT(*)
SI_UNIT(.CENTI.,.METRE.)
);
#9816=(
NAMED_UNIT(*)
PLANE_ANGLE_UNIT()
SI_UNIT($,.RADIAN.)
);
#9817=(
NAMED_UNIT(*)
SI_UNIT($,.STERADIAN.)
SOLID_ANGLE_UNIT()
);
#9847=SHAPE_DEFINITION_REPRESENTATION(#9920,#9964);
#9920=PRODUCT_DEFINITION_SHAPE('',$,#10000);
#9964=SHAPE_REPRESENTATION('',(#5634),#9807);
#9970=PRODUCT_DEFINITION_CONTEXT('part definition',#10077,'design');
#10000=PRODUCT_DEFINITION('Moving leaf and hinge pin',
'Moving leaf and hinge pin',#10035,#9970);
#10035=PRODUCT_DEFINITION_FORMATION('',$,#10108);
#10077=APPLICATION_CONTEXT(
'Core Data for Automotive Mechanical Design Process');
#10078=PRODUCT_CONTEXT('part definition',#10077,'mechanical');
#10108=PRODUCT('Moving leaf and hinge pin','Moving leaf and hinge pin',
'Moving leaf and hinge pin',(#10078));
#10177=COLOUR_RGB('Grey',0.48,0.52,0.57);
#10178=FILL_AREA_STYLE_COLOUR('',#10177);
#10179=FILL_AREA_STYLE('',(#10178));
#10180=SURFACE_STYLE_FILL_AREA(#10179);
#10181=SURFACE_SIDE_STYLE('',(#10180));
#10182=SURFACE_STYLE_USAGE(.BOTH.,#10181);
#10183=PRESENTATION_STYLE_ASSIGNMENT((#10182));
ENDSEC;
END-ISO-10303-21;
